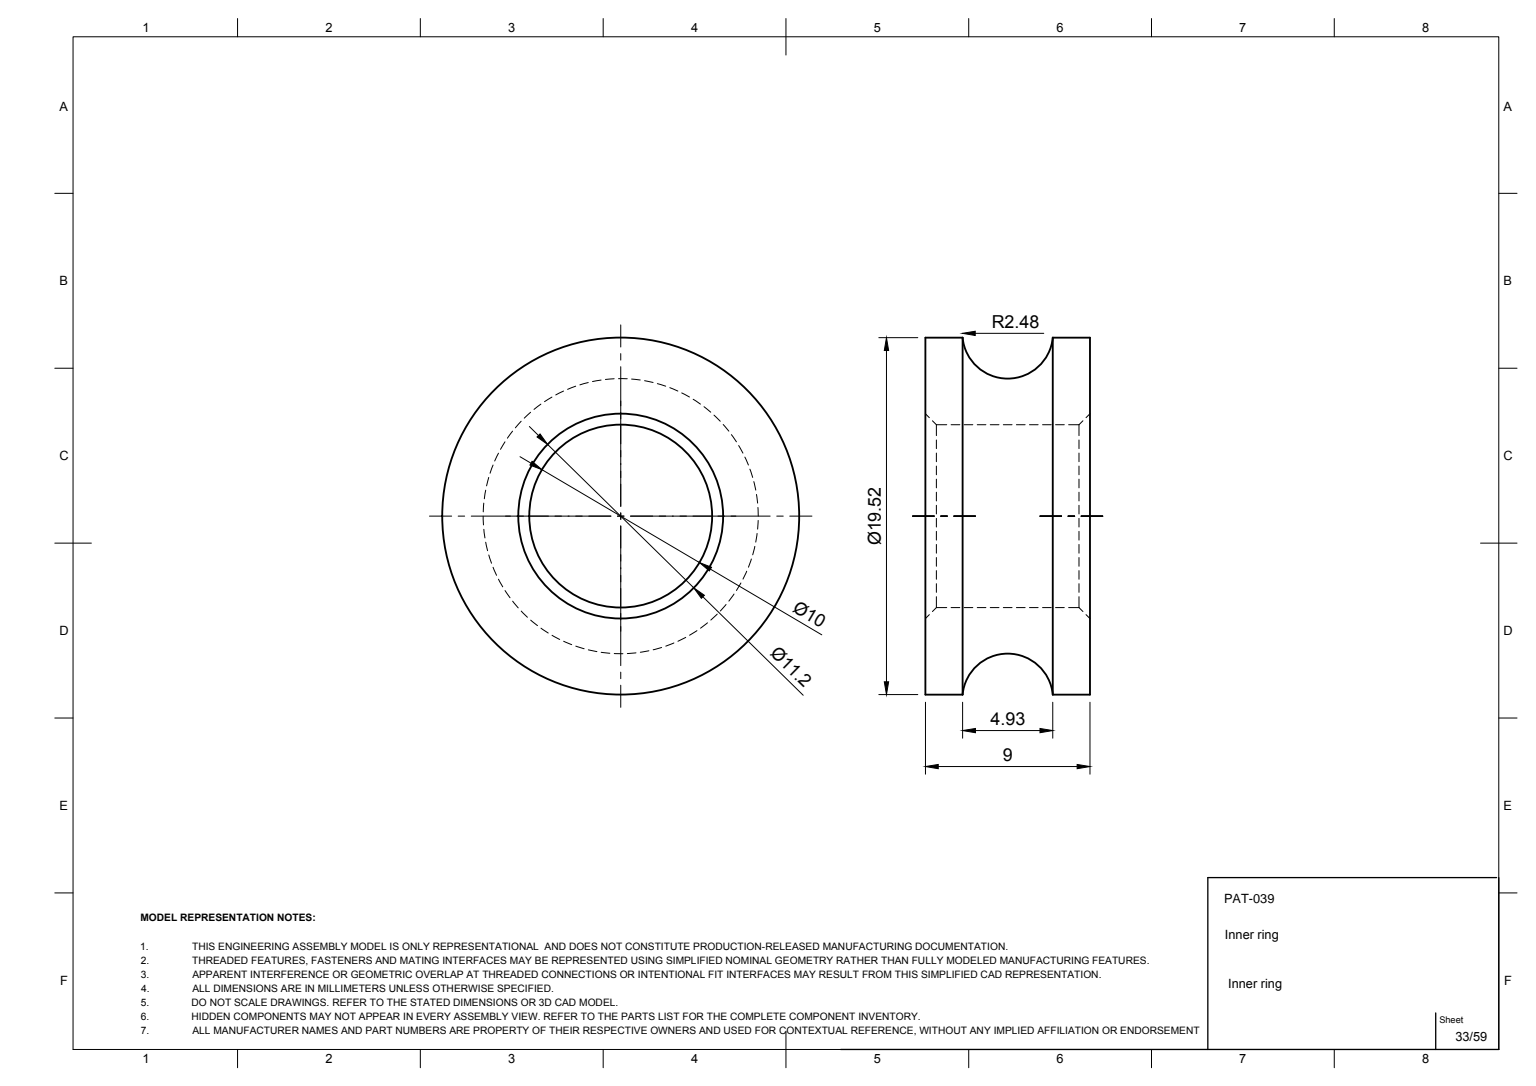
ISO-10303-21;
HEADER;
/* Generated by software containing ST-Developer
 * from STEP Tools, Inc. (www.steptools.com) 
 */

FILE_DESCRIPTION(
/* description */ ('Four-bar parallelogram arm'),
/* implementation_level */ '2;1');

FILE_NAME(
/* name */ 'Inner ring.step',
/* time_stamp */ '2026-10-28T03:24:55-07:00',
/* author */ (''),
/* organization */ (''),
/* preprocessor_version */ 'ST-DEVELOPER v20.2',
/* originating_system */ 'Autodesk Translation Framework v15.17.0.0',
/* authorisation */ '');

FILE_SCHEMA (('AUTOMOTIVE_DESIGN { 1 0 10303 214 3 1 1 }'));
ENDSEC;

DATA;
#10=MECHANICAL_DESIGN_GEOMETRIC_PRESENTATION_REPRESENTATION('',(#654),#14512);
#475=TOROIDAL_SURFACE('',#8508,1.,0.247676);
#480=CONICAL_SURFACE('',#8519,0.53,0.785398163397448);
#481=CONICAL_SURFACE('',#8526,0.53,0.785398163397448);
#554=SHAPE_REPRESENTATION_RELATIONSHIP('SRR','None',#14778,#604);
#604=ADVANCED_BREP_SHAPE_REPRESENTATION('',(#711),#14493);
#654=STYLED_ITEM('',(#15087),#711);
#711=MANIFOLD_SOLID_BREP('Body1',#7359);
#937=FACE_BOUND('',#2087,.T.);
#938=FACE_BOUND('',#2090,.T.);
#1127=PLANE('',#8521);
#1128=PLANE('',#8524);
#1460=FACE_OUTER_BOUND('',#2082,.T.);
#1461=FACE_OUTER_BOUND('',#2083,.T.);
#1462=FACE_OUTER_BOUND('',#2084,.T.);
#1463=FACE_OUTER_BOUND('',#2085,.T.);
#1464=FACE_OUTER_BOUND('',#2086,.T.);
#1465=FACE_OUTER_BOUND('',#2088,.T.);
#1466=FACE_OUTER_BOUND('',#2089,.T.);
#1467=FACE_OUTER_BOUND('',#2091,.T.);
#2082=EDGE_LOOP('',(#6084,#6085,#6086,#6087,#6088,#6089));
#2083=EDGE_LOOP('',(#6090,#6091,#6092,#6093,#6094));
#2084=EDGE_LOOP('',(#6095,#6096,#6097,#6098));
#2085=EDGE_LOOP('',(#6099,#6100,#6101,#6102));
#2086=EDGE_LOOP('',(#6103));
#2087=EDGE_LOOP('',(#6104));
#2088=EDGE_LOOP('',(#6105,#6106,#6107,#6108,#6109));
#2089=EDGE_LOOP('',(#6110));
#2090=EDGE_LOOP('',(#6111));
#2091=EDGE_LOOP('',(#6112,#6113,#6114,#6115));
#2580=LINE('',#13250,#2974);
#2581=LINE('',#13256,#2975);
#2582=LINE('',#13260,#2976);
#2583=LINE('',#13266,#2977);
#2584=LINE('',#13271,#2978);
#2974=VECTOR('',#10392,0.976185);
#2975=VECTOR('',#10399,0.5);
#2976=VECTOR('',#10404,0.53);
#2977=VECTOR('',#10413,0.976185);
#2978=VECTOR('',#10420,0.53);
#3374=CIRCLE('',#8509,0.976185);
#3375=CIRCLE('',#8510,0.976185);
#3376=CIRCLE('',#8511,0.247676);
#3377=CIRCLE('',#8512,0.976185);
#3378=CIRCLE('',#8513,0.976185);
#3379=CIRCLE('',#8515,0.976185);
#3380=CIRCLE('',#8517,0.5);
#3381=CIRCLE('',#8518,0.5);
#3382=CIRCLE('',#8520,0.56);
#3383=CIRCLE('',#8523,0.976185);
#3384=CIRCLE('',#8525,0.56);
#3908=VERTEX_POINT('',#13239);
#3909=VERTEX_POINT('',#13240);
#3910=VERTEX_POINT('',#13243);
#3911=VERTEX_POINT('',#13245);
#3912=VERTEX_POINT('',#13249);
#3913=VERTEX_POINT('',#13253);
#3914=VERTEX_POINT('',#13255);
#3915=VERTEX_POINT('',#13259);
#3916=VERTEX_POINT('',#13264);
#3917=VERTEX_POINT('',#13268);
#4673=EDGE_CURVE('',#3908,#3909,#3374,.T.);
#4674=EDGE_CURVE('',#3909,#3908,#3375,.T.);
#4675=EDGE_CURVE('',#3909,#3910,#3376,.T.);
#4676=EDGE_CURVE('',#3911,#3910,#3377,.T.);
#4677=EDGE_CURVE('',#3910,#3911,#3378,.T.);
#4678=EDGE_CURVE('',#3911,#3912,#2580,.T.);
#4679=EDGE_CURVE('',#3912,#3912,#3379,.T.);
#4680=EDGE_CURVE('',#3913,#3913,#3380,.T.);
#4681=EDGE_CURVE('',#3913,#3914,#2581,.T.);
#4682=EDGE_CURVE('',#3914,#3914,#3381,.T.);
#4683=EDGE_CURVE('',#3914,#3915,#2582,.T.);
#4684=EDGE_CURVE('',#3915,#3915,#3382,.T.);
#4685=EDGE_CURVE('',#3916,#3916,#3383,.T.);
#4686=EDGE_CURVE('',#3916,#3908,#2583,.T.);
#4687=EDGE_CURVE('',#3917,#3917,#3384,.T.);
#4688=EDGE_CURVE('',#3917,#3913,#2584,.T.);
#6084=ORIENTED_EDGE('',*,*,#4673,.F.);
#6085=ORIENTED_EDGE('',*,*,#4674,.F.);
#6086=ORIENTED_EDGE('',*,*,#4675,.T.);
#6087=ORIENTED_EDGE('',*,*,#4676,.F.);
#6088=ORIENTED_EDGE('',*,*,#4677,.F.);
#6089=ORIENTED_EDGE('',*,*,#4675,.F.);
#6090=ORIENTED_EDGE('',*,*,#4676,.T.);
#6091=ORIENTED_EDGE('',*,*,#4677,.T.);
#6092=ORIENTED_EDGE('',*,*,#4678,.T.);
#6093=ORIENTED_EDGE('',*,*,#4679,.T.);
#6094=ORIENTED_EDGE('',*,*,#4678,.F.);
#6095=ORIENTED_EDGE('',*,*,#4680,.T.);
#6096=ORIENTED_EDGE('',*,*,#4681,.T.);
#6097=ORIENTED_EDGE('',*,*,#4682,.F.);
#6098=ORIENTED_EDGE('',*,*,#4681,.F.);
#6099=ORIENTED_EDGE('',*,*,#4682,.T.);
#6100=ORIENTED_EDGE('',*,*,#4683,.T.);
#6101=ORIENTED_EDGE('',*,*,#4684,.F.);
#6102=ORIENTED_EDGE('',*,*,#4683,.F.);
#6103=ORIENTED_EDGE('',*,*,#4679,.F.);
#6104=ORIENTED_EDGE('',*,*,#4684,.T.);
#6105=ORIENTED_EDGE('',*,*,#4685,.F.);
#6106=ORIENTED_EDGE('',*,*,#4686,.T.);
#6107=ORIENTED_EDGE('',*,*,#4673,.T.);
#6108=ORIENTED_EDGE('',*,*,#4674,.T.);
#6109=ORIENTED_EDGE('',*,*,#4686,.F.);
#6110=ORIENTED_EDGE('',*,*,#4685,.T.);
#6111=ORIENTED_EDGE('',*,*,#4687,.F.);
#6112=ORIENTED_EDGE('',*,*,#4687,.T.);
#6113=ORIENTED_EDGE('',*,*,#4688,.T.);
#6114=ORIENTED_EDGE('',*,*,#4680,.F.);
#6115=ORIENTED_EDGE('',*,*,#4688,.F.);
#6848=CYLINDRICAL_SURFACE('',#8514,0.976185);
#6849=CYLINDRICAL_SURFACE('',#8516,0.5);
#6850=CYLINDRICAL_SURFACE('',#8522,0.976185);
#7165=ADVANCED_FACE('',(#1460),#475,.F.);
#7166=ADVANCED_FACE('',(#1461),#6848,.T.);
#7167=ADVANCED_FACE('',(#1462),#6849,.F.);
#7168=ADVANCED_FACE('',(#1463),#480,.F.);
#7169=ADVANCED_FACE('',(#1464,#937),#1127,.T.);
#7170=ADVANCED_FACE('',(#1465),#6850,.T.);
#7171=ADVANCED_FACE('',(#1466,#938),#1128,.T.);
#7172=ADVANCED_FACE('',(#1467),#481,.F.);
#7359=CLOSED_SHELL('',(#7165,#7166,#7167,#7168,#7169,#7170,#7171,#7172));
#8507=AXIS2_PLACEMENT_3D('',#13237,#10376,#10377);
#8508=AXIS2_PLACEMENT_3D('',#13238,#10378,#10379);
#8509=AXIS2_PLACEMENT_3D('',#13241,#10380,#10381);
#8510=AXIS2_PLACEMENT_3D('',#13242,#10382,#10383);
#8511=AXIS2_PLACEMENT_3D('',#13244,#10384,#10385);
#8512=AXIS2_PLACEMENT_3D('',#13246,#10386,#10387);
#8513=AXIS2_PLACEMENT_3D('',#13247,#10388,#10389);
#8514=AXIS2_PLACEMENT_3D('',#13248,#10390,#10391);
#8515=AXIS2_PLACEMENT_3D('',#13251,#10393,#10394);
#8516=AXIS2_PLACEMENT_3D('',#13252,#10395,#10396);
#8517=AXIS2_PLACEMENT_3D('',#13254,#10397,#10398);
#8518=AXIS2_PLACEMENT_3D('',#13257,#10400,#10401);
#8519=AXIS2_PLACEMENT_3D('',#13258,#10402,#10403);
#8520=AXIS2_PLACEMENT_3D('',#13261,#10405,#10406);
#8521=AXIS2_PLACEMENT_3D('',#13262,#10407,#10408);
#8522=AXIS2_PLACEMENT_3D('',#13263,#10409,#10410);
#8523=AXIS2_PLACEMENT_3D('',#13265,#10411,#10412);
#8524=AXIS2_PLACEMENT_3D('',#13267,#10414,#10415);
#8525=AXIS2_PLACEMENT_3D('',#13269,#10416,#10417);
#8526=AXIS2_PLACEMENT_3D('',#13270,#10418,#10419);
#10376=DIRECTION('axis',(0.,0.,1.));
#10377=DIRECTION('refdir',(1.,0.,0.));
#10378=DIRECTION('center_axis',(0.,-1.,0.));
#10379=DIRECTION('ref_axis',(0.,0.,-1.));
#10380=DIRECTION('center_axis',(0.,-1.,0.));
#10381=DIRECTION('ref_axis',(1.,0.,0.));
#10382=DIRECTION('center_axis',(0.,-1.,0.));
#10383=DIRECTION('ref_axis',(1.,0.,0.));
#10384=DIRECTION('center_axis',(1.,0.,1.22464679914735E-16));
#10385=DIRECTION('ref_axis',(-1.22464679914735E-16,0.,1.));
#10386=DIRECTION('center_axis',(0.,1.,0.));
#10387=DIRECTION('ref_axis',(1.,0.,0.));
#10388=DIRECTION('center_axis',(0.,1.,0.));
#10389=DIRECTION('ref_axis',(1.,0.,0.));
#10390=DIRECTION('center_axis',(0.,-1.,0.));
#10391=DIRECTION('ref_axis',(1.,0.,0.));
#10392=DIRECTION('',(0.,1.,0.));
#10393=DIRECTION('center_axis',(0.,-1.,0.));
#10394=DIRECTION('ref_axis',(1.,0.,0.));
#10395=DIRECTION('center_axis',(0.,-1.,0.));
#10396=DIRECTION('ref_axis',(1.,0.,0.));
#10397=DIRECTION('center_axis',(0.,-1.,0.));
#10398=DIRECTION('ref_axis',(1.,0.,0.));
#10399=DIRECTION('',(0.,1.,0.));
#10400=DIRECTION('center_axis',(0.,-1.,0.));
#10401=DIRECTION('ref_axis',(1.,0.,0.));
#10402=DIRECTION('center_axis',(0.,1.,0.));
#10403=DIRECTION('ref_axis',(1.,0.,0.));
#10404=DIRECTION('',(-0.707106781186547,0.707106781186548,-8.65956056235493E-17));
#10405=DIRECTION('center_axis',(0.,-1.,0.));
#10406=DIRECTION('ref_axis',(1.,0.,0.));
#10407=DIRECTION('center_axis',(0.,1.,0.));
#10408=DIRECTION('ref_axis',(0.,0.,1.));
#10409=DIRECTION('center_axis',(0.,-1.,0.));
#10410=DIRECTION('ref_axis',(1.,0.,0.));
#10411=DIRECTION('center_axis',(0.,-1.,0.));
#10412=DIRECTION('ref_axis',(1.,0.,0.));
#10413=DIRECTION('',(0.,1.,0.));
#10414=DIRECTION('center_axis',(0.,-1.,0.));
#10415=DIRECTION('ref_axis',(0.,0.,-1.));
#10416=DIRECTION('center_axis',(0.,-1.,0.));
#10417=DIRECTION('ref_axis',(1.,0.,0.));
#10418=DIRECTION('center_axis',(0.,-1.,0.));
#10419=DIRECTION('ref_axis',(1.,0.,0.));
#10420=DIRECTION('',(0.707106781186547,0.707106781186548,8.65956056235493E-17));
#13237=CARTESIAN_POINT('',(0.,0.,0.));
#13238=CARTESIAN_POINT('Origin',(0.,0.,0.));
#13239=CARTESIAN_POINT('',(-0.976185,-0.246528389340863,-1.19548183562566E-16));
#13240=CARTESIAN_POINT('',(-1.19548183562566E-16,-0.246528389340863,0.976185));
#13241=CARTESIAN_POINT('Origin',(0.,-0.246528389340863,0.));
#13242=CARTESIAN_POINT('Origin',(0.,-0.246528389340863,0.));
#13243=CARTESIAN_POINT('',(-1.19548183562566E-16,0.246528389340863,0.976185));
#13244=CARTESIAN_POINT('Origin',(-1.22464679914735E-16,0.,1.));
#13245=CARTESIAN_POINT('',(-0.976185,0.246528389340863,1.19548183562566E-16));
#13246=CARTESIAN_POINT('Origin',(0.,0.246528389340863,0.));
#13247=CARTESIAN_POINT('Origin',(0.,0.246528389340863,0.));
#13248=CARTESIAN_POINT('Origin',(0.,0.,0.));
#13249=CARTESIAN_POINT('',(-0.976185,0.45,-1.19548183562566E-16));
#13250=CARTESIAN_POINT('',(-0.976185,0.,-1.19548183562566E-16));
#13251=CARTESIAN_POINT('Origin',(0.,0.45,0.));
#13252=CARTESIAN_POINT('Origin',(0.,0.,0.));
#13253=CARTESIAN_POINT('',(-0.5,-0.39,-6.12323399573677E-17));
#13254=CARTESIAN_POINT('Origin',(0.,-0.39,0.));
#13255=CARTESIAN_POINT('',(-0.5,0.39,-6.12323399573677E-17));
#13256=CARTESIAN_POINT('',(-0.5,0.,-6.12323399573677E-17));
#13257=CARTESIAN_POINT('Origin',(0.,0.39,0.));
#13258=CARTESIAN_POINT('Origin',(0.,0.42,0.));
#13259=CARTESIAN_POINT('',(-0.56,0.45,-6.85802207522518E-17));
#13260=CARTESIAN_POINT('',(-0.53,0.42,-6.49062803548097E-17));
#13261=CARTESIAN_POINT('Origin',(0.,0.45,0.));
#13262=CARTESIAN_POINT('Origin',(0.976185,0.45,0.));
#13263=CARTESIAN_POINT('Origin',(0.,0.,0.));
#13264=CARTESIAN_POINT('',(-0.976185,-0.45,-1.19548183562566E-16));
#13265=CARTESIAN_POINT('Origin',(0.,-0.45,0.));
#13266=CARTESIAN_POINT('',(-0.976185,0.,-1.19548183562566E-16));
#13267=CARTESIAN_POINT('Origin',(0.56,-0.45,0.));
#13268=CARTESIAN_POINT('',(-0.56,-0.45,-6.85802207522518E-17));
#13269=CARTESIAN_POINT('Origin',(0.,-0.45,0.));
#13270=CARTESIAN_POINT('Origin',(0.,-0.42,0.));
#13271=CARTESIAN_POINT('',(-0.53,-0.42,-6.49062803548097E-17));
#14436=UNCERTAINTY_MEASURE_WITH_UNIT(LENGTH_MEASURE(0.001),#14513,
'DISTANCE_ACCURACY_VALUE',
'Maximum model space distance between geometric entities at asserted c
onnectivities');
#14455=UNCERTAINTY_MEASURE_WITH_UNIT(LENGTH_MEASURE(0.001),#14513,
'DISTANCE_ACCURACY_VALUE',
'Maximum model space distance between geometric entities at asserted c
onnectivities');
#14493=(
GEOMETRIC_REPRESENTATION_CONTEXT(3)
GLOBAL_UNCERTAINTY_ASSIGNED_CONTEXT((#14436))
GLOBAL_UNIT_ASSIGNED_CONTEXT((#14513,#14515,#14516))
REPRESENTATION_CONTEXT('','3D')
);
#14512=(
GEOMETRIC_REPRESENTATION_CONTEXT(3)
GLOBAL_UNCERTAINTY_ASSIGNED_CONTEXT((#14455))
GLOBAL_UNIT_ASSIGNED_CONTEXT((#14513,#14515,#14516))
REPRESENTATION_CONTEXT('','3D')
);
#14513=(
LENGTH_UNIT()
NAMED_UNIT(*)
SI_UNIT(.CENTI.,.METRE.)
);
#14515=(
NAMED_UNIT(*)
PLANE_ANGLE_UNIT()
SI_UNIT($,.RADIAN.)
);
#14516=(
NAMED_UNIT(*)
SI_UNIT($,.STERADIAN.)
SOLID_ANGLE_UNIT()
);
#14554=SHAPE_DEFINITION_REPRESENTATION(#14610,#14778);
#14610=PRODUCT_DEFINITION_SHAPE('',$,#14835);
#14778=SHAPE_REPRESENTATION('',(#8507),#14493);
#14797=PRODUCT_DEFINITION_CONTEXT('part definition',#14967,'design');
#14835=PRODUCT_DEFINITION('Inner ring','Inner ring',#14891,#14797);
#14891=PRODUCT_DEFINITION_FORMATION('',$,#15006);
#14967=APPLICATION_CONTEXT(
'Core Data for Automotive Mechanical Design Process');
#14968=PRODUCT_CONTEXT('part definition',#14967,'mechanical');
#15006=PRODUCT('Inner ring','Inner ring','Inner ring',(#14968));
#15081=COLOUR_RGB('Grey',0.48,0.52,0.57);
#15082=FILL_AREA_STYLE_COLOUR('',#15081);
#15083=FILL_AREA_STYLE('',(#15082));
#15084=SURFACE_STYLE_FILL_AREA(#15083);
#15085=SURFACE_SIDE_STYLE('',(#15084));
#15086=SURFACE_STYLE_USAGE(.BOTH.,#15085);
#15087=PRESENTATION_STYLE_ASSIGNMENT((#15086));
ENDSEC;
END-ISO-10303-21;
